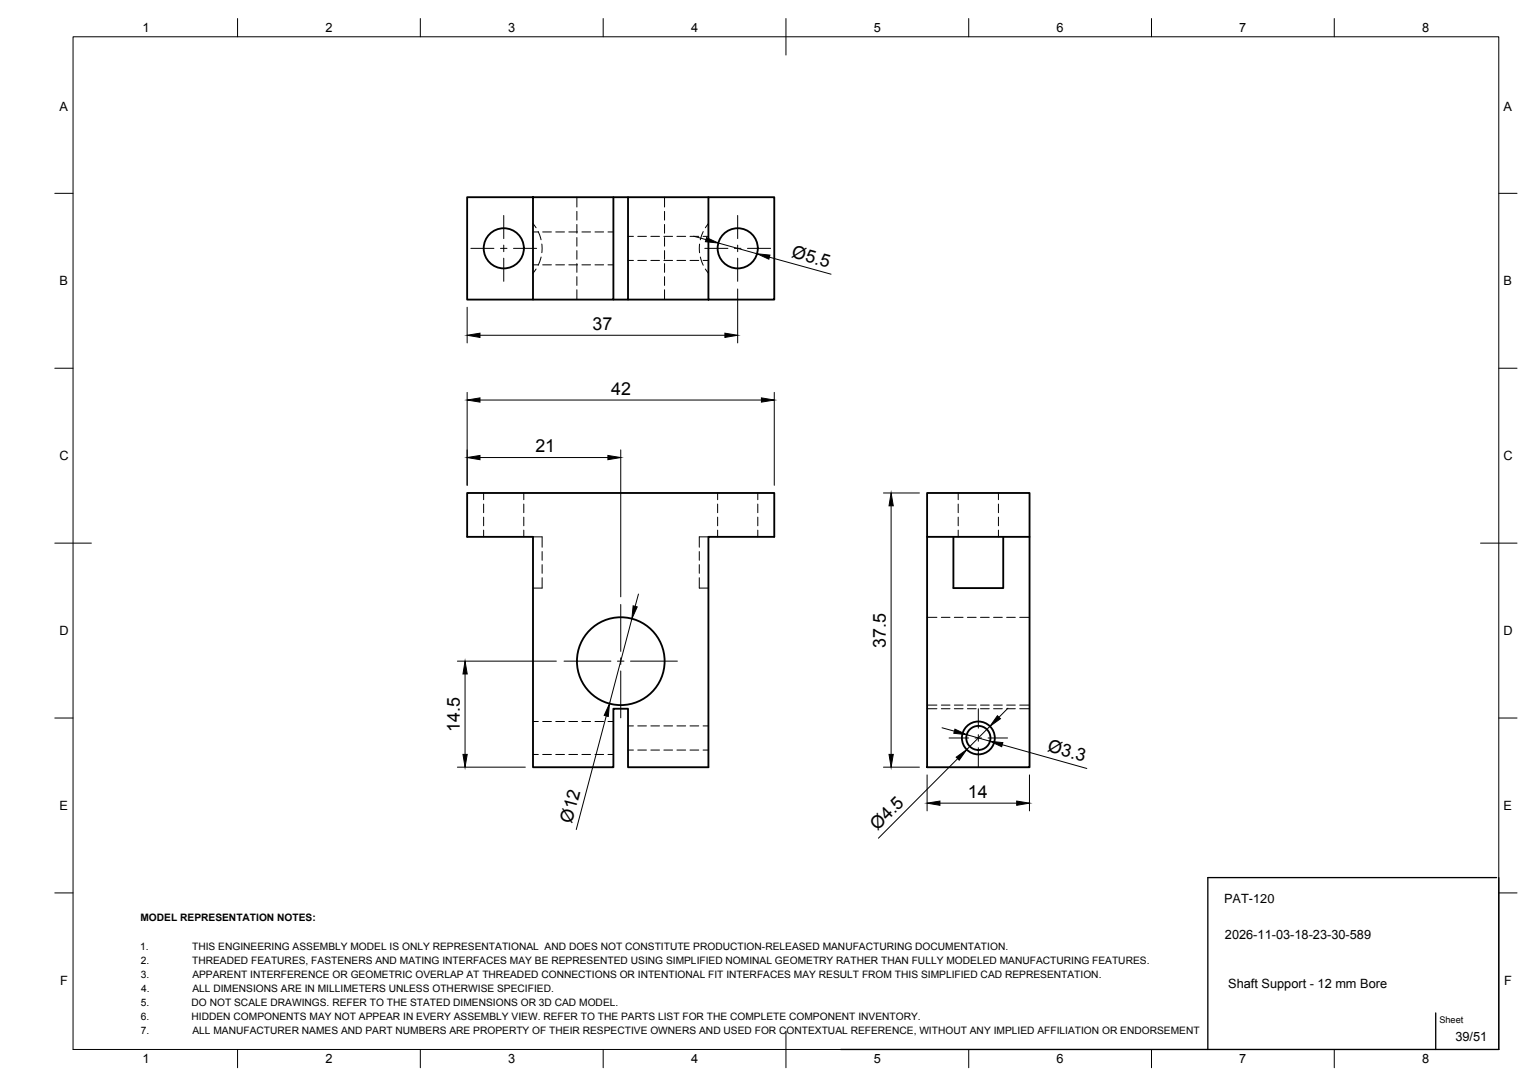
ISO-10303-21;
HEADER;
/* Generated by software containing ST-Developer
 * from STEP Tools, Inc. (www.steptools.com) 
 */

FILE_DESCRIPTION(
/* description */ ('Vibration shaker table dummy'),
/* implementation_level */ '2;1');

FILE_NAME(
/* name */ 'Shaft Support - 12 mm Bore.step',
/* time_stamp */ '2026-10-27T10:55:14-07:00',
/* author */ (''),
/* organization */ (''),
/* preprocessor_version */ 'ST-DEVELOPER v20.2',
/* originating_system */ 'Autodesk Translation Framework v15.17.0.0',
/* authorisation */ '');

FILE_SCHEMA (('AUTOMOTIVE_DESIGN { 1 0 10303 214 3 1 1 }'));
ENDSEC;

DATA;
#10=MECHANICAL_DESIGN_GEOMETRIC_PRESENTATION_REPRESENTATION('',(#720),#22394);
#628=SHAPE_REPRESENTATION_RELATIONSHIP('SRR','None',#22674,#674);
#674=ADVANCED_BREP_SHAPE_REPRESENTATION('',(#766),#22380);
#720=STYLED_ITEM('',(#22961),#766);
#766=MANIFOLD_SOLID_BREP('Body1',#9238);
#947=FACE_BOUND('',#2313,.T.);
#948=FACE_BOUND('',#2315,.T.);
#949=FACE_BOUND('',#2317,.T.);
#950=FACE_BOUND('',#2324,.T.);
#951=FACE_BOUND('',#2327,.T.);
#952=FACE_BOUND('',#2328,.T.);
#953=FACE_BOUND('',#2331,.T.);
#954=FACE_BOUND('',#2334,.T.);
#955=FACE_BOUND('',#2337,.T.);
#956=FACE_BOUND('',#2340,.T.);
#1234=PLANE('',#10350);
#1235=PLANE('',#10357);
#1236=PLANE('',#10358);
#1237=PLANE('',#10360);
#1238=PLANE('',#10362);
#1239=PLANE('',#10376);
#1240=PLANE('',#10377);
#1241=PLANE('',#10378);
#1242=PLANE('',#10379);
#1243=PLANE('',#10380);
#1244=PLANE('',#10381);
#1245=PLANE('',#10382);
#1246=PLANE('',#10383);
#1247=PLANE('',#10384);
#1248=PLANE('',#10385);
#1249=PLANE('',#10386);
#1638=FACE_OUTER_BOUND('',#2308,.T.);
#1639=FACE_OUTER_BOUND('',#2309,.T.);
#1640=FACE_OUTER_BOUND('',#2310,.T.);
#1641=FACE_OUTER_BOUND('',#2311,.T.);
#1642=FACE_OUTER_BOUND('',#2312,.T.);
#1643=FACE_OUTER_BOUND('',#2314,.T.);
#1644=FACE_OUTER_BOUND('',#2316,.T.);
#1645=FACE_OUTER_BOUND('',#2318,.T.);
#1646=FACE_OUTER_BOUND('',#2319,.T.);
#1647=FACE_OUTER_BOUND('',#2320,.T.);
#1648=FACE_OUTER_BOUND('',#2321,.T.);
#1649=FACE_OUTER_BOUND('',#2322,.T.);
#1650=FACE_OUTER_BOUND('',#2323,.T.);
#1651=FACE_OUTER_BOUND('',#2325,.T.);
#1652=FACE_OUTER_BOUND('',#2326,.T.);
#1653=FACE_OUTER_BOUND('',#2329,.T.);
#1654=FACE_OUTER_BOUND('',#2330,.T.);
#1655=FACE_OUTER_BOUND('',#2332,.T.);
#1656=FACE_OUTER_BOUND('',#2333,.T.);
#1657=FACE_OUTER_BOUND('',#2335,.T.);
#1658=FACE_OUTER_BOUND('',#2336,.T.);
#1659=FACE_OUTER_BOUND('',#2338,.T.);
#1660=FACE_OUTER_BOUND('',#2339,.T.);
#2308=EDGE_LOOP('',(#7508,#7509));
#2309=EDGE_LOOP('',(#7510,#7511,#7512,#7513));
#2310=EDGE_LOOP('',(#7514,#7515,#7516,#7517));
#2311=EDGE_LOOP('',(#7518,#7519));
#2312=EDGE_LOOP('',(#7520,#7521,#7522,#7523,#7524,#7525));
#2313=EDGE_LOOP('',(#7526));
#2314=EDGE_LOOP('',(#7527,#7528,#7529,#7530,#7531,#7532,#7533,#7534));
#2315=EDGE_LOOP('',(#7535));
#2316=EDGE_LOOP('',(#7536,#7537,#7538,#7539,#7540,#7541));
#2317=EDGE_LOOP('',(#7542));
#2318=EDGE_LOOP('',(#7543,#7544,#7545,#7546));
#2319=EDGE_LOOP('',(#7547,#7548,#7549,#7550));
#2320=EDGE_LOOP('',(#7551,#7552,#7553,#7554));
#2321=EDGE_LOOP('',(#7555,#7556,#7557,#7558));
#2322=EDGE_LOOP('',(#7559,#7560,#7561,#7562));
#2323=EDGE_LOOP('',(#7563,#7564,#7565,#7566,#7567,#7568,#7569,#7570,#7571,
#7572,#7573,#7574));
#2324=EDGE_LOOP('',(#7575));
#2325=EDGE_LOOP('',(#7576,#7577,#7578,#7579));
#2326=EDGE_LOOP('',(#7580,#7581,#7582,#7583));
#2327=EDGE_LOOP('',(#7584));
#2328=EDGE_LOOP('',(#7585));
#2329=EDGE_LOOP('',(#7586,#7587,#7588,#7589));
#2330=EDGE_LOOP('',(#7590,#7591,#7592,#7593,#7594,#7595,#7596,#7597));
#2331=EDGE_LOOP('',(#7598));
#2332=EDGE_LOOP('',(#7599,#7600,#7601,#7602));
#2333=EDGE_LOOP('',(#7603,#7604,#7605,#7606));
#2334=EDGE_LOOP('',(#7607));
#2335=EDGE_LOOP('',(#7608,#7609,#7610,#7611));
#2336=EDGE_LOOP('',(#7612,#7613,#7614,#7615));
#2337=EDGE_LOOP('',(#7616));
#2338=EDGE_LOOP('',(#7617,#7618,#7619,#7620));
#2339=EDGE_LOOP('',(#7621,#7622,#7623,#7624,#7625,#7626,#7627,#7628,#7629,
#7630,#7631,#7632));
#2340=EDGE_LOOP('',(#7633));
#2989=LINE('',#21115,#3608);
#2990=LINE('',#21119,#3609);
#2991=LINE('',#21122,#3610);
#2992=LINE('',#21126,#3611);
#2993=LINE('',#21130,#3612);
#2994=LINE('',#21133,#3613);
#2995=LINE('',#21136,#3614);
#2996=LINE('',#21138,#3615);
#2997=LINE('',#21140,#3616);
#2998=LINE('',#21142,#3617);
#2999=LINE('',#21143,#3618);
#3000=LINE('',#21148,#3619);
#3001=LINE('',#21150,#3620);
#3002=LINE('',#21151,#3621);
#3003=LINE('',#21157,#3622);
#3004=LINE('',#21159,#3623);
#3005=LINE('',#21160,#3624);
#3006=LINE('',#21162,#3625);
#3007=LINE('',#21163,#3626);
#3008=LINE('',#21170,#3627);
#3009=LINE('',#21174,#3628);
#3010=LINE('',#21179,#3629);
#3011=LINE('',#21183,#3630);
#3012=LINE('',#21188,#3631);
#3013=LINE('',#21192,#3632);
#3014=LINE('',#21194,#3633);
#3015=LINE('',#21195,#3634);
#3016=LINE('',#21197,#3635);
#3017=LINE('',#21199,#3636);
#3018=LINE('',#21201,#3637);
#3019=LINE('',#21203,#3638);
#3020=LINE('',#21205,#3639);
#3021=LINE('',#21206,#3640);
#3022=LINE('',#21209,#3641);
#3023=LINE('',#21210,#3642);
#3024=LINE('',#21213,#3643);
#3025=LINE('',#21214,#3644);
#3026=LINE('',#21216,#3645);
#3027=LINE('',#21219,#3646);
#3028=LINE('',#21220,#3647);
#3029=LINE('',#21223,#3648);
#3030=LINE('',#21224,#3649);
#3031=LINE('',#21227,#3650);
#3032=LINE('',#21228,#3651);
#3033=LINE('',#21231,#3652);
#3034=LINE('',#21232,#3653);
#3035=LINE('',#21235,#3654);
#3036=LINE('',#21236,#3655);
#3037=LINE('',#21238,#3656);
#3608=VECTOR('',#12499,1.);
#3609=VECTOR('',#12504,1.);
#3610=VECTOR('',#12507,1.);
#3611=VECTOR('',#12510,1.);
#3612=VECTOR('',#12513,1.);
#3613=VECTOR('',#12518,1.);
#3614=VECTOR('',#12521,1.);
#3615=VECTOR('',#12522,1.);
#3616=VECTOR('',#12523,1.);
#3617=VECTOR('',#12524,1.);
#3618=VECTOR('',#12525,1.);
#3619=VECTOR('',#12530,1.);
#3620=VECTOR('',#12531,1.);
#3621=VECTOR('',#12532,1.);
#3622=VECTOR('',#12537,1.);
#3623=VECTOR('',#12538,1.);
#3624=VECTOR('',#12539,1.);
#3625=VECTOR('',#12540,1.);
#3626=VECTOR('',#12541,1.);
#3627=VECTOR('',#12548,0.225);
#3628=VECTOR('',#12553,0.165);
#3629=VECTOR('',#12560,0.275);
#3630=VECTOR('',#12565,0.275);
#3631=VECTOR('',#12570,0.6);
#3632=VECTOR('',#12575,1.);
#3633=VECTOR('',#12576,1.);
#3634=VECTOR('',#12577,1.);
#3635=VECTOR('',#12578,1.);
#3636=VECTOR('',#12579,1.);
#3637=VECTOR('',#12580,1.);
#3638=VECTOR('',#12581,1.);
#3639=VECTOR('',#12582,1.);
#3640=VECTOR('',#12583,1.);
#3641=VECTOR('',#12586,1.);
#3642=VECTOR('',#12587,1.);
#3643=VECTOR('',#12590,1.);
#3644=VECTOR('',#12591,1.);
#3645=VECTOR('',#12594,1.);
#3646=VECTOR('',#12597,1.);
#3647=VECTOR('',#12598,1.);
#3648=VECTOR('',#12601,1.);
#3649=VECTOR('',#12602,1.);
#3650=VECTOR('',#12605,1.);
#3651=VECTOR('',#12606,1.);
#3652=VECTOR('',#12609,1.);
#3653=VECTOR('',#12610,1.);
#3654=VECTOR('',#12613,1.);
#3655=VECTOR('',#12614,1.);
#3656=VECTOR('',#12617,1.);
#4120=CIRCLE('',#10351,0.525);
#4121=CIRCLE('',#10353,0.525);
#4122=CIRCLE('',#10355,0.525);
#4123=CIRCLE('',#10356,0.525);
#4124=CIRCLE('',#10359,0.275);
#4125=CIRCLE('',#10361,0.165);
#4126=CIRCLE('',#10363,0.275);
#4127=CIRCLE('',#10365,0.225);
#4128=CIRCLE('',#10366,0.225);
#4129=CIRCLE('',#10368,0.165);
#4130=CIRCLE('',#10370,0.275);
#4131=CIRCLE('',#10372,0.275);
#4132=CIRCLE('',#10374,0.6);
#4133=CIRCLE('',#10375,0.6);
#4787=VERTEX_POINT('',#21113);
#4788=VERTEX_POINT('',#21114);
#4789=VERTEX_POINT('',#21118);
#4790=VERTEX_POINT('',#21120);
#4791=VERTEX_POINT('',#21124);
#4792=VERTEX_POINT('',#21125);
#4793=VERTEX_POINT('',#21127);
#4794=VERTEX_POINT('',#21129);
#4795=VERTEX_POINT('',#21135);
#4796=VERTEX_POINT('',#21137);
#4797=VERTEX_POINT('',#21139);
#4798=VERTEX_POINT('',#21141);
#4799=VERTEX_POINT('',#21144);
#4800=VERTEX_POINT('',#21147);
#4801=VERTEX_POINT('',#21149);
#4802=VERTEX_POINT('',#21152);
#4803=VERTEX_POINT('',#21155);
#4804=VERTEX_POINT('',#21156);
#4805=VERTEX_POINT('',#21158);
#4806=VERTEX_POINT('',#21161);
#4807=VERTEX_POINT('',#21164);
#4808=VERTEX_POINT('',#21167);
#4809=VERTEX_POINT('',#21169);
#4810=VERTEX_POINT('',#21173);
#4811=VERTEX_POINT('',#21177);
#4812=VERTEX_POINT('',#21181);
#4813=VERTEX_POINT('',#21185);
#4814=VERTEX_POINT('',#21187);
#4815=VERTEX_POINT('',#21191);
#4816=VERTEX_POINT('',#21193);
#4817=VERTEX_POINT('',#21196);
#4818=VERTEX_POINT('',#21198);
#4819=VERTEX_POINT('',#21200);
#4820=VERTEX_POINT('',#21202);
#4821=VERTEX_POINT('',#21204);
#4822=VERTEX_POINT('',#21208);
#4823=VERTEX_POINT('',#21212);
#4824=VERTEX_POINT('',#21218);
#4825=VERTEX_POINT('',#21222);
#4826=VERTEX_POINT('',#21226);
#4827=VERTEX_POINT('',#21230);
#4828=VERTEX_POINT('',#21234);
#5747=EDGE_CURVE('',#4787,#4788,#2989,.T.);
#5748=EDGE_CURVE('',#4788,#4787,#4120,.T.);
#5749=EDGE_CURVE('',#4789,#4787,#2990,.T.);
#5750=EDGE_CURVE('',#4790,#4789,#4121,.T.);
#5751=EDGE_CURVE('',#4788,#4790,#2991,.T.);
#5752=EDGE_CURVE('',#4791,#4792,#2992,.T.);
#5753=EDGE_CURVE('',#4791,#4793,#4122,.T.);
#5754=EDGE_CURVE('',#4794,#4793,#2993,.T.);
#5755=EDGE_CURVE('',#4792,#4794,#4123,.T.);
#5756=EDGE_CURVE('',#4793,#4791,#2994,.T.);
#5757=EDGE_CURVE('',#4789,#4795,#2995,.T.);
#5758=EDGE_CURVE('',#4796,#4795,#2996,.T.);
#5759=EDGE_CURVE('',#4796,#4797,#2997,.T.);
#5760=EDGE_CURVE('',#4798,#4797,#2998,.T.);
#5761=EDGE_CURVE('',#4798,#4790,#2999,.T.);
#5762=EDGE_CURVE('',#4799,#4799,#4124,.T.);
#5763=EDGE_CURVE('',#4800,#4798,#3000,.T.);
#5764=EDGE_CURVE('',#4800,#4801,#3001,.T.);
#5765=EDGE_CURVE('',#4795,#4801,#3002,.T.);
#5766=EDGE_CURVE('',#4802,#4802,#4125,.T.);
#5767=EDGE_CURVE('',#4803,#4804,#3003,.T.);
#5768=EDGE_CURVE('',#4805,#4804,#3004,.T.);
#5769=EDGE_CURVE('',#4792,#4805,#3005,.T.);
#5770=EDGE_CURVE('',#4806,#4794,#3006,.T.);
#5771=EDGE_CURVE('',#4803,#4806,#3007,.T.);
#5772=EDGE_CURVE('',#4807,#4807,#4126,.T.);
#5773=EDGE_CURVE('',#4808,#4808,#4127,.T.);
#5774=EDGE_CURVE('',#4808,#4809,#3008,.T.);
#5775=EDGE_CURVE('',#4809,#4809,#4128,.T.);
#5776=EDGE_CURVE('',#4802,#4810,#3009,.T.);
#5777=EDGE_CURVE('',#4810,#4810,#4129,.T.);
#5778=EDGE_CURVE('',#4811,#4811,#4130,.T.);
#5779=EDGE_CURVE('',#4811,#4799,#3010,.T.);
#5780=EDGE_CURVE('',#4812,#4812,#4131,.T.);
#5781=EDGE_CURVE('',#4812,#4807,#3011,.T.);
#5782=EDGE_CURVE('',#4813,#4813,#4132,.T.);
#5783=EDGE_CURVE('',#4813,#4814,#3012,.T.);
#5784=EDGE_CURVE('',#4814,#4814,#4133,.T.);
#5785=EDGE_CURVE('',#4797,#4815,#3013,.T.);
#5786=EDGE_CURVE('',#4815,#4816,#3014,.T.);
#5787=EDGE_CURVE('',#4816,#4803,#3015,.T.);
#5788=EDGE_CURVE('',#4806,#4817,#3016,.T.);
#5789=EDGE_CURVE('',#4817,#4818,#3017,.T.);
#5790=EDGE_CURVE('',#4818,#4819,#3018,.T.);
#5791=EDGE_CURVE('',#4819,#4820,#3019,.T.);
#5792=EDGE_CURVE('',#4820,#4821,#3020,.T.);
#5793=EDGE_CURVE('',#4821,#4800,#3021,.T.);
#5794=EDGE_CURVE('',#4822,#4796,#3022,.T.);
#5795=EDGE_CURVE('',#4815,#4822,#3023,.T.);
#5796=EDGE_CURVE('',#4823,#4822,#3024,.T.);
#5797=EDGE_CURVE('',#4816,#4823,#3025,.T.);
#5798=EDGE_CURVE('',#4804,#4823,#3026,.T.);
#5799=EDGE_CURVE('',#4824,#4805,#3027,.T.);
#5800=EDGE_CURVE('',#4817,#4824,#3028,.T.);
#5801=EDGE_CURVE('',#4825,#4824,#3029,.T.);
#5802=EDGE_CURVE('',#4818,#4825,#3030,.T.);
#5803=EDGE_CURVE('',#4826,#4825,#3031,.T.);
#5804=EDGE_CURVE('',#4819,#4826,#3032,.T.);
#5805=EDGE_CURVE('',#4827,#4826,#3033,.T.);
#5806=EDGE_CURVE('',#4820,#4827,#3034,.T.);
#5807=EDGE_CURVE('',#4828,#4827,#3035,.T.);
#5808=EDGE_CURVE('',#4821,#4828,#3036,.T.);
#5809=EDGE_CURVE('',#4801,#4828,#3037,.T.);
#7508=ORIENTED_EDGE('',*,*,#5747,.F.);
#7509=ORIENTED_EDGE('',*,*,#5748,.F.);
#7510=ORIENTED_EDGE('',*,*,#5749,.F.);
#7511=ORIENTED_EDGE('',*,*,#5750,.F.);
#7512=ORIENTED_EDGE('',*,*,#5751,.F.);
#7513=ORIENTED_EDGE('',*,*,#5748,.T.);
#7514=ORIENTED_EDGE('',*,*,#5752,.F.);
#7515=ORIENTED_EDGE('',*,*,#5753,.T.);
#7516=ORIENTED_EDGE('',*,*,#5754,.F.);
#7517=ORIENTED_EDGE('',*,*,#5755,.F.);
#7518=ORIENTED_EDGE('',*,*,#5756,.F.);
#7519=ORIENTED_EDGE('',*,*,#5753,.F.);
#7520=ORIENTED_EDGE('',*,*,#5757,.T.);
#7521=ORIENTED_EDGE('',*,*,#5758,.F.);
#7522=ORIENTED_EDGE('',*,*,#5759,.T.);
#7523=ORIENTED_EDGE('',*,*,#5760,.F.);
#7524=ORIENTED_EDGE('',*,*,#5761,.T.);
#7525=ORIENTED_EDGE('',*,*,#5750,.T.);
#7526=ORIENTED_EDGE('',*,*,#5762,.T.);
#7527=ORIENTED_EDGE('',*,*,#5749,.T.);
#7528=ORIENTED_EDGE('',*,*,#5747,.T.);
#7529=ORIENTED_EDGE('',*,*,#5751,.T.);
#7530=ORIENTED_EDGE('',*,*,#5761,.F.);
#7531=ORIENTED_EDGE('',*,*,#5763,.F.);
#7532=ORIENTED_EDGE('',*,*,#5764,.T.);
#7533=ORIENTED_EDGE('',*,*,#5765,.F.);
#7534=ORIENTED_EDGE('',*,*,#5757,.F.);
#7535=ORIENTED_EDGE('',*,*,#5766,.T.);
#7536=ORIENTED_EDGE('',*,*,#5767,.T.);
#7537=ORIENTED_EDGE('',*,*,#5768,.F.);
#7538=ORIENTED_EDGE('',*,*,#5769,.F.);
#7539=ORIENTED_EDGE('',*,*,#5755,.T.);
#7540=ORIENTED_EDGE('',*,*,#5770,.F.);
#7541=ORIENTED_EDGE('',*,*,#5771,.F.);
#7542=ORIENTED_EDGE('',*,*,#5772,.T.);
#7543=ORIENTED_EDGE('',*,*,#5773,.F.);
#7544=ORIENTED_EDGE('',*,*,#5774,.T.);
#7545=ORIENTED_EDGE('',*,*,#5775,.F.);
#7546=ORIENTED_EDGE('',*,*,#5774,.F.);
#7547=ORIENTED_EDGE('',*,*,#5766,.F.);
#7548=ORIENTED_EDGE('',*,*,#5776,.T.);
#7549=ORIENTED_EDGE('',*,*,#5777,.F.);
#7550=ORIENTED_EDGE('',*,*,#5776,.F.);
#7551=ORIENTED_EDGE('',*,*,#5778,.F.);
#7552=ORIENTED_EDGE('',*,*,#5779,.T.);
#7553=ORIENTED_EDGE('',*,*,#5762,.F.);
#7554=ORIENTED_EDGE('',*,*,#5779,.F.);
#7555=ORIENTED_EDGE('',*,*,#5780,.F.);
#7556=ORIENTED_EDGE('',*,*,#5781,.T.);
#7557=ORIENTED_EDGE('',*,*,#5772,.F.);
#7558=ORIENTED_EDGE('',*,*,#5781,.F.);
#7559=ORIENTED_EDGE('',*,*,#5782,.F.);
#7560=ORIENTED_EDGE('',*,*,#5783,.T.);
#7561=ORIENTED_EDGE('',*,*,#5784,.F.);
#7562=ORIENTED_EDGE('',*,*,#5783,.F.);
#7563=ORIENTED_EDGE('',*,*,#5760,.T.);
#7564=ORIENTED_EDGE('',*,*,#5785,.T.);
#7565=ORIENTED_EDGE('',*,*,#5786,.T.);
#7566=ORIENTED_EDGE('',*,*,#5787,.T.);
#7567=ORIENTED_EDGE('',*,*,#5771,.T.);
#7568=ORIENTED_EDGE('',*,*,#5788,.T.);
#7569=ORIENTED_EDGE('',*,*,#5789,.T.);
#7570=ORIENTED_EDGE('',*,*,#5790,.T.);
#7571=ORIENTED_EDGE('',*,*,#5791,.T.);
#7572=ORIENTED_EDGE('',*,*,#5792,.T.);
#7573=ORIENTED_EDGE('',*,*,#5793,.T.);
#7574=ORIENTED_EDGE('',*,*,#5763,.T.);
#7575=ORIENTED_EDGE('',*,*,#5782,.T.);
#7576=ORIENTED_EDGE('',*,*,#5759,.F.);
#7577=ORIENTED_EDGE('',*,*,#5794,.F.);
#7578=ORIENTED_EDGE('',*,*,#5795,.F.);
#7579=ORIENTED_EDGE('',*,*,#5785,.F.);
#7580=ORIENTED_EDGE('',*,*,#5795,.T.);
#7581=ORIENTED_EDGE('',*,*,#5796,.F.);
#7582=ORIENTED_EDGE('',*,*,#5797,.F.);
#7583=ORIENTED_EDGE('',*,*,#5786,.F.);
#7584=ORIENTED_EDGE('',*,*,#5778,.T.);
#7585=ORIENTED_EDGE('',*,*,#5780,.T.);
#7586=ORIENTED_EDGE('',*,*,#5797,.T.);
#7587=ORIENTED_EDGE('',*,*,#5798,.F.);
#7588=ORIENTED_EDGE('',*,*,#5767,.F.);
#7589=ORIENTED_EDGE('',*,*,#5787,.F.);
#7590=ORIENTED_EDGE('',*,*,#5752,.T.);
#7591=ORIENTED_EDGE('',*,*,#5769,.T.);
#7592=ORIENTED_EDGE('',*,*,#5799,.F.);
#7593=ORIENTED_EDGE('',*,*,#5800,.F.);
#7594=ORIENTED_EDGE('',*,*,#5788,.F.);
#7595=ORIENTED_EDGE('',*,*,#5770,.T.);
#7596=ORIENTED_EDGE('',*,*,#5754,.T.);
#7597=ORIENTED_EDGE('',*,*,#5756,.T.);
#7598=ORIENTED_EDGE('',*,*,#5775,.T.);
#7599=ORIENTED_EDGE('',*,*,#5800,.T.);
#7600=ORIENTED_EDGE('',*,*,#5801,.F.);
#7601=ORIENTED_EDGE('',*,*,#5802,.F.);
#7602=ORIENTED_EDGE('',*,*,#5789,.F.);
#7603=ORIENTED_EDGE('',*,*,#5802,.T.);
#7604=ORIENTED_EDGE('',*,*,#5803,.F.);
#7605=ORIENTED_EDGE('',*,*,#5804,.F.);
#7606=ORIENTED_EDGE('',*,*,#5790,.F.);
#7607=ORIENTED_EDGE('',*,*,#5773,.T.);
#7608=ORIENTED_EDGE('',*,*,#5804,.T.);
#7609=ORIENTED_EDGE('',*,*,#5805,.F.);
#7610=ORIENTED_EDGE('',*,*,#5806,.F.);
#7611=ORIENTED_EDGE('',*,*,#5791,.F.);
#7612=ORIENTED_EDGE('',*,*,#5806,.T.);
#7613=ORIENTED_EDGE('',*,*,#5807,.F.);
#7614=ORIENTED_EDGE('',*,*,#5808,.F.);
#7615=ORIENTED_EDGE('',*,*,#5792,.F.);
#7616=ORIENTED_EDGE('',*,*,#5777,.T.);
#7617=ORIENTED_EDGE('',*,*,#5808,.T.);
#7618=ORIENTED_EDGE('',*,*,#5809,.F.);
#7619=ORIENTED_EDGE('',*,*,#5764,.F.);
#7620=ORIENTED_EDGE('',*,*,#5793,.F.);
#7621=ORIENTED_EDGE('',*,*,#5758,.T.);
#7622=ORIENTED_EDGE('',*,*,#5765,.T.);
#7623=ORIENTED_EDGE('',*,*,#5809,.T.);
#7624=ORIENTED_EDGE('',*,*,#5807,.T.);
#7625=ORIENTED_EDGE('',*,*,#5805,.T.);
#7626=ORIENTED_EDGE('',*,*,#5803,.T.);
#7627=ORIENTED_EDGE('',*,*,#5801,.T.);
#7628=ORIENTED_EDGE('',*,*,#5799,.T.);
#7629=ORIENTED_EDGE('',*,*,#5768,.T.);
#7630=ORIENTED_EDGE('',*,*,#5798,.T.);
#7631=ORIENTED_EDGE('',*,*,#5796,.T.);
#7632=ORIENTED_EDGE('',*,*,#5794,.T.);
#7633=ORIENTED_EDGE('',*,*,#5784,.T.);
#8623=CYLINDRICAL_SURFACE('',#10352,0.525);
#8624=CYLINDRICAL_SURFACE('',#10354,0.525);
#8625=CYLINDRICAL_SURFACE('',#10364,0.225);
#8626=CYLINDRICAL_SURFACE('',#10367,0.165);
#8627=CYLINDRICAL_SURFACE('',#10369,0.275);
#8628=CYLINDRICAL_SURFACE('',#10371,0.275);
#8629=CYLINDRICAL_SURFACE('',#10373,0.6);
#9003=ADVANCED_FACE('',(#1638),#1234,.F.);
#9004=ADVANCED_FACE('',(#1639),#8623,.F.);
#9005=ADVANCED_FACE('',(#1640),#8624,.F.);
#9006=ADVANCED_FACE('',(#1641),#1235,.F.);
#9007=ADVANCED_FACE('',(#1642,#947),#1236,.T.);
#9008=ADVANCED_FACE('',(#1643,#948),#1237,.T.);
#9009=ADVANCED_FACE('',(#1644,#949),#1238,.T.);
#9010=ADVANCED_FACE('',(#1645),#8625,.F.);
#9011=ADVANCED_FACE('',(#1646),#8626,.F.);
#9012=ADVANCED_FACE('',(#1647),#8627,.F.);
#9013=ADVANCED_FACE('',(#1648),#8628,.F.);
#9014=ADVANCED_FACE('',(#1649),#8629,.F.);
#9015=ADVANCED_FACE('',(#1650,#950),#1239,.T.);
#9016=ADVANCED_FACE('',(#1651),#1240,.T.);
#9017=ADVANCED_FACE('',(#1652,#951,#952),#1241,.T.);
#9018=ADVANCED_FACE('',(#1653),#1242,.T.);
#9019=ADVANCED_FACE('',(#1654,#953),#1243,.T.);
#9020=ADVANCED_FACE('',(#1655),#1244,.T.);
#9021=ADVANCED_FACE('',(#1656,#954),#1245,.T.);
#9022=ADVANCED_FACE('',(#1657),#1246,.T.);
#9023=ADVANCED_FACE('',(#1658,#955),#1247,.T.);
#9024=ADVANCED_FACE('',(#1659),#1248,.T.);
#9025=ADVANCED_FACE('',(#1660,#956),#1249,.T.);
#9238=CLOSED_SHELL('',(#9003,#9004,#9005,#9006,#9007,#9008,#9009,#9010,
#9011,#9012,#9013,#9014,#9015,#9016,#9017,#9018,#9019,#9020,#9021,#9022,
#9023,#9024,#9025));
#10349=AXIS2_PLACEMENT_3D('',#21111,#12495,#12496);
#10350=AXIS2_PLACEMENT_3D('',#21112,#12497,#12498);
#10351=AXIS2_PLACEMENT_3D('',#21116,#12500,#12501);
#10352=AXIS2_PLACEMENT_3D('',#21117,#12502,#12503);
#10353=AXIS2_PLACEMENT_3D('',#21121,#12505,#12506);
#10354=AXIS2_PLACEMENT_3D('',#21123,#12508,#12509);
#10355=AXIS2_PLACEMENT_3D('',#21128,#12511,#12512);
#10356=AXIS2_PLACEMENT_3D('',#21131,#12514,#12515);
#10357=AXIS2_PLACEMENT_3D('',#21132,#12516,#12517);
#10358=AXIS2_PLACEMENT_3D('',#21134,#12519,#12520);
#10359=AXIS2_PLACEMENT_3D('',#21145,#12526,#12527);
#10360=AXIS2_PLACEMENT_3D('',#21146,#12528,#12529);
#10361=AXIS2_PLACEMENT_3D('',#21153,#12533,#12534);
#10362=AXIS2_PLACEMENT_3D('',#21154,#12535,#12536);
#10363=AXIS2_PLACEMENT_3D('',#21165,#12542,#12543);
#10364=AXIS2_PLACEMENT_3D('',#21166,#12544,#12545);
#10365=AXIS2_PLACEMENT_3D('',#21168,#12546,#12547);
#10366=AXIS2_PLACEMENT_3D('',#21171,#12549,#12550);
#10367=AXIS2_PLACEMENT_3D('',#21172,#12551,#12552);
#10368=AXIS2_PLACEMENT_3D('',#21175,#12554,#12555);
#10369=AXIS2_PLACEMENT_3D('',#21176,#12556,#12557);
#10370=AXIS2_PLACEMENT_3D('',#21178,#12558,#12559);
#10371=AXIS2_PLACEMENT_3D('',#21180,#12561,#12562);
#10372=AXIS2_PLACEMENT_3D('',#21182,#12563,#12564);
#10373=AXIS2_PLACEMENT_3D('',#21184,#12566,#12567);
#10374=AXIS2_PLACEMENT_3D('',#21186,#12568,#12569);
#10375=AXIS2_PLACEMENT_3D('',#21189,#12571,#12572);
#10376=AXIS2_PLACEMENT_3D('',#21190,#12573,#12574);
#10377=AXIS2_PLACEMENT_3D('',#21207,#12584,#12585);
#10378=AXIS2_PLACEMENT_3D('',#21211,#12588,#12589);
#10379=AXIS2_PLACEMENT_3D('',#21215,#12592,#12593);
#10380=AXIS2_PLACEMENT_3D('',#21217,#12595,#12596);
#10381=AXIS2_PLACEMENT_3D('',#21221,#12599,#12600);
#10382=AXIS2_PLACEMENT_3D('',#21225,#12603,#12604);
#10383=AXIS2_PLACEMENT_3D('',#21229,#12607,#12608);
#10384=AXIS2_PLACEMENT_3D('',#21233,#12611,#12612);
#10385=AXIS2_PLACEMENT_3D('',#21237,#12615,#12616);
#10386=AXIS2_PLACEMENT_3D('',#21239,#12618,#12619);
#12495=DIRECTION('axis',(0.,0.,1.));
#12496=DIRECTION('refdir',(1.,0.,0.));
#12497=DIRECTION('center_axis',(0.,0.,1.));
#12498=DIRECTION('ref_axis',(1.,0.,0.));
#12499=DIRECTION('',(0.,-1.,0.));
#12500=DIRECTION('center_axis',(0.,0.,1.));
#12501=DIRECTION('ref_axis',(1.,0.,0.));
#12502=DIRECTION('center_axis',(0.,0.,1.));
#12503=DIRECTION('ref_axis',(1.,0.,0.));
#12504=DIRECTION('',(0.,0.,1.));
#12505=DIRECTION('center_axis',(0.,0.,1.));
#12506=DIRECTION('ref_axis',(1.,0.,0.));
#12507=DIRECTION('',(0.,0.,-1.));
#12508=DIRECTION('center_axis',(0.,0.,1.));
#12509=DIRECTION('ref_axis',(-1.,1.22464679914735E-16,0.));
#12510=DIRECTION('',(0.,0.,-1.));
#12511=DIRECTION('center_axis',(0.,0.,1.));
#12512=DIRECTION('ref_axis',(1.,0.,0.));
#12513=DIRECTION('',(0.,0.,1.));
#12514=DIRECTION('center_axis',(0.,0.,1.));
#12515=DIRECTION('ref_axis',(1.,0.,0.));
#12516=DIRECTION('center_axis',(0.,0.,1.));
#12517=DIRECTION('ref_axis',(1.,0.,0.));
#12518=DIRECTION('',(0.,1.,0.));
#12519=DIRECTION('center_axis',(0.,0.,1.));
#12520=DIRECTION('ref_axis',(1.,0.,0.));
#12521=DIRECTION('',(0.,1.,0.));
#12522=DIRECTION('',(1.,0.,0.));
#12523=DIRECTION('',(0.,-1.,0.));
#12524=DIRECTION('',(-1.,0.,0.));
#12525=DIRECTION('',(0.,1.,0.));
#12526=DIRECTION('center_axis',(0.,0.,-1.));
#12527=DIRECTION('ref_axis',(1.,0.,0.));
#12528=DIRECTION('center_axis',(-1.,0.,0.));
#12529=DIRECTION('ref_axis',(0.,0.,1.));
#12530=DIRECTION('',(0.,0.,-1.));
#12531=DIRECTION('',(0.,1.,0.));
#12532=DIRECTION('',(0.,0.,1.));
#12533=DIRECTION('center_axis',(1.,0.,0.));
#12534=DIRECTION('ref_axis',(0.,0.,-1.));
#12535=DIRECTION('center_axis',(0.,0.,1.));
#12536=DIRECTION('ref_axis',(1.,0.,0.));
#12537=DIRECTION('',(0.,1.,0.));
#12538=DIRECTION('',(1.,0.,0.));
#12539=DIRECTION('',(0.,1.,0.));
#12540=DIRECTION('',(0.,1.,0.));
#12541=DIRECTION('',(-1.,0.,0.));
#12542=DIRECTION('center_axis',(0.,0.,-1.));
#12543=DIRECTION('ref_axis',(1.,0.,0.));
#12544=DIRECTION('center_axis',(1.,0.,0.));
#12545=DIRECTION('ref_axis',(0.,0.,-1.));
#12546=DIRECTION('center_axis',(1.,0.,0.));
#12547=DIRECTION('ref_axis',(0.,0.,-1.));
#12548=DIRECTION('',(1.,0.,0.));
#12549=DIRECTION('center_axis',(-1.,0.,0.));
#12550=DIRECTION('ref_axis',(0.,0.,-1.));
#12551=DIRECTION('center_axis',(1.,0.,0.));
#12552=DIRECTION('ref_axis',(0.,0.,-1.));
#12553=DIRECTION('',(1.,0.,0.));
#12554=DIRECTION('center_axis',(-1.,0.,0.));
#12555=DIRECTION('ref_axis',(0.,0.,-1.));
#12556=DIRECTION('center_axis',(0.,0.,1.));
#12557=DIRECTION('ref_axis',(1.,0.,0.));
#12558=DIRECTION('center_axis',(0.,0.,1.));
#12559=DIRECTION('ref_axis',(1.,0.,0.));
#12560=DIRECTION('',(0.,0.,1.));
#12561=DIRECTION('center_axis',(0.,0.,1.));
#12562=DIRECTION('ref_axis',(1.,0.,0.));
#12563=DIRECTION('center_axis',(0.,0.,1.));
#12564=DIRECTION('ref_axis',(1.,0.,0.));
#12565=DIRECTION('',(0.,0.,1.));
#12566=DIRECTION('center_axis',(0.,1.,0.));
#12567=DIRECTION('ref_axis',(1.,0.,0.));
#12568=DIRECTION('center_axis',(0.,1.,0.));
#12569=DIRECTION('ref_axis',(1.,0.,0.));
#12570=DIRECTION('',(0.,1.,0.));
#12571=DIRECTION('center_axis',(0.,-1.,0.));
#12572=DIRECTION('ref_axis',(1.,0.,0.));
#12573=DIRECTION('center_axis',(0.,-1.,0.));
#12574=DIRECTION('ref_axis',(0.,0.,-1.));
#12575=DIRECTION('',(0.,0.,-1.));
#12576=DIRECTION('',(1.,0.,0.));
#12577=DIRECTION('',(0.,0.,1.));
#12578=DIRECTION('',(0.,0.,1.));
#12579=DIRECTION('',(-1.,0.,0.));
#12580=DIRECTION('',(0.,0.,-1.));
#12581=DIRECTION('',(-1.,0.,0.));
#12582=DIRECTION('',(0.,0.,1.));
#12583=DIRECTION('',(-1.,0.,0.));
#12584=DIRECTION('center_axis',(-1.,0.,0.));
#12585=DIRECTION('ref_axis',(0.,0.,1.));
#12586=DIRECTION('',(0.,0.,1.));
#12587=DIRECTION('',(0.,1.,0.));
#12588=DIRECTION('center_axis',(0.,0.,-1.));
#12589=DIRECTION('ref_axis',(-1.,0.,0.));
#12590=DIRECTION('',(-1.,0.,0.));
#12591=DIRECTION('',(0.,1.,0.));
#12592=DIRECTION('center_axis',(1.,0.,0.));
#12593=DIRECTION('ref_axis',(0.,0.,-1.));
#12594=DIRECTION('',(0.,0.,-1.));
#12595=DIRECTION('center_axis',(1.,0.,0.));
#12596=DIRECTION('ref_axis',(0.,0.,-1.));
#12597=DIRECTION('',(0.,0.,-1.));
#12598=DIRECTION('',(0.,1.,0.));
#12599=DIRECTION('center_axis',(0.,0.,1.));
#12600=DIRECTION('ref_axis',(1.,0.,0.));
#12601=DIRECTION('',(1.,0.,0.));
#12602=DIRECTION('',(0.,1.,0.));
#12603=DIRECTION('center_axis',(-1.,0.,0.));
#12604=DIRECTION('ref_axis',(0.,0.,1.));
#12605=DIRECTION('',(0.,0.,1.));
#12606=DIRECTION('',(0.,1.,0.));
#12607=DIRECTION('center_axis',(0.,0.,1.));
#12608=DIRECTION('ref_axis',(1.,0.,0.));
#12609=DIRECTION('',(1.,0.,0.));
#12610=DIRECTION('',(0.,1.,0.));
#12611=DIRECTION('center_axis',(1.,0.,0.));
#12612=DIRECTION('ref_axis',(0.,0.,-1.));
#12613=DIRECTION('',(0.,0.,-1.));
#12614=DIRECTION('',(0.,1.,0.));
#12615=DIRECTION('center_axis',(0.,0.,1.));
#12616=DIRECTION('ref_axis',(1.,0.,0.));
#12617=DIRECTION('',(1.,0.,0.));
#12618=DIRECTION('center_axis',(0.,1.,0.));
#12619=DIRECTION('ref_axis',(0.,0.,1.));
#21111=CARTESIAN_POINT('',(0.,0.,0.));
#21112=CARTESIAN_POINT('Origin',(-1.6,0.,1.3));
#21113=CARTESIAN_POINT('',(-1.2,0.340036762718386,1.3));
#21114=CARTESIAN_POINT('',(-1.2,-0.340036762718386,1.3));
#21115=CARTESIAN_POINT('',(-1.2,0.,1.3));
#21116=CARTESIAN_POINT('Origin',(-1.6,0.,1.3));
#21117=CARTESIAN_POINT('Origin',(-1.6,0.,0.6));
#21118=CARTESIAN_POINT('',(-1.2,0.340036762718386,0.6));
#21119=CARTESIAN_POINT('',(-1.2,0.340036762718386,0.6));
#21120=CARTESIAN_POINT('',(-1.2,-0.340036762718386,0.6));
#21121=CARTESIAN_POINT('Origin',(-1.6,0.,0.6));
#21122=CARTESIAN_POINT('',(-1.2,-0.340036762718386,0.6));
#21123=CARTESIAN_POINT('Origin',(1.6,0.,0.6));
#21124=CARTESIAN_POINT('',(1.2,0.340036762718386,1.3));
#21125=CARTESIAN_POINT('',(1.2,0.340036762718386,0.6));
#21126=CARTESIAN_POINT('',(1.2,0.340036762718386,0.6));
#21127=CARTESIAN_POINT('',(1.2,-0.340036762718386,1.3));
#21128=CARTESIAN_POINT('Origin',(1.6,0.,1.3));
#21129=CARTESIAN_POINT('',(1.2,-0.340036762718386,0.6));
#21130=CARTESIAN_POINT('',(1.2,-0.340036762718386,0.6));
#21131=CARTESIAN_POINT('Origin',(1.6,0.,0.6));
#21132=CARTESIAN_POINT('Origin',(1.6,0.,1.3));
#21133=CARTESIAN_POINT('',(1.2,0.,1.3));
#21134=CARTESIAN_POINT('Origin',(-2.1,0.,0.6));
#21135=CARTESIAN_POINT('',(-1.2,0.7,0.6));
#21136=CARTESIAN_POINT('',(-1.2,0.,0.6));
#21137=CARTESIAN_POINT('',(-2.1,0.7,0.6));
#21138=CARTESIAN_POINT('',(-1.2,0.7,0.6));
#21139=CARTESIAN_POINT('',(-2.1,-0.7,0.6));
#21140=CARTESIAN_POINT('',(-2.1,0.,0.6));
#21141=CARTESIAN_POINT('',(-1.2,-0.7,0.6));
#21142=CARTESIAN_POINT('',(-1.2,-0.7,0.6));
#21143=CARTESIAN_POINT('',(-1.2,0.,0.6));
#21144=CARTESIAN_POINT('',(-1.875,3.36777869765522E-17,0.6));
#21145=CARTESIAN_POINT('Origin',(-1.6,0.,0.6));
#21146=CARTESIAN_POINT('Origin',(-1.2,0.,0.6));
#21147=CARTESIAN_POINT('',(-1.2,-0.7,3.75));
#21148=CARTESIAN_POINT('',(-1.2,-0.7,3.75));
#21149=CARTESIAN_POINT('',(-1.2,0.7,3.75));
#21150=CARTESIAN_POINT('',(-1.2,0.,3.75));
#21151=CARTESIAN_POINT('',(-1.2,0.7,3.75));
#21152=CARTESIAN_POINT('',(-1.2,-2.02066721859313E-17,3.515));
#21153=CARTESIAN_POINT('Origin',(-1.2,0.,3.35));
#21154=CARTESIAN_POINT('Origin',(1.2,0.,0.6));
#21155=CARTESIAN_POINT('',(2.1,-0.7,0.6));
#21156=CARTESIAN_POINT('',(2.1,0.7,0.6));
#21157=CARTESIAN_POINT('',(2.1,0.,0.6));
#21158=CARTESIAN_POINT('',(1.2,0.7,0.6));
#21159=CARTESIAN_POINT('',(2.1,0.7,0.6));
#21160=CARTESIAN_POINT('',(1.2,0.,0.6));
#21161=CARTESIAN_POINT('',(1.2,-0.7,0.6));
#21162=CARTESIAN_POINT('',(1.2,0.,0.6));
#21163=CARTESIAN_POINT('',(2.1,-0.7,0.6));
#21164=CARTESIAN_POINT('',(1.325,3.36777869765522E-17,0.6));
#21165=CARTESIAN_POINT('Origin',(1.6,0.,0.6));
#21166=CARTESIAN_POINT('Origin',(0.1,0.,3.35));
#21167=CARTESIAN_POINT('',(0.1,-2.75545529808155E-17,3.575));
#21168=CARTESIAN_POINT('Origin',(0.1,0.,3.35));
#21169=CARTESIAN_POINT('',(1.2,2.75545529808155E-17,3.575));
#21170=CARTESIAN_POINT('',(0.1,-2.75545529808155E-17,3.575));
#21171=CARTESIAN_POINT('Origin',(1.2,0.,3.35));
#21172=CARTESIAN_POINT('Origin',(0.,0.,3.35));
#21173=CARTESIAN_POINT('',(-0.1,2.02066721859313E-17,3.515));
#21174=CARTESIAN_POINT('',(0.,-2.02066721859313E-17,3.515));
#21175=CARTESIAN_POINT('Origin',(-0.1,0.,3.35));
#21176=CARTESIAN_POINT('Origin',(-1.6,0.,-0.05));
#21177=CARTESIAN_POINT('',(-1.875,-3.36777869765522E-17,0.));
#21178=CARTESIAN_POINT('Origin',(-1.6,0.,0.));
#21179=CARTESIAN_POINT('',(-1.875,-3.36777869765522E-17,-0.05));
#21180=CARTESIAN_POINT('Origin',(1.6,0.,-0.05));
#21181=CARTESIAN_POINT('',(1.325,-3.36777869765522E-17,0.));
#21182=CARTESIAN_POINT('Origin',(1.6,0.,0.));
#21183=CARTESIAN_POINT('',(1.325,-3.36777869765522E-17,-0.05));
#21184=CARTESIAN_POINT('Origin',(0.,0.,2.3));
#21185=CARTESIAN_POINT('',(-0.6,-0.7,2.3));
#21186=CARTESIAN_POINT('Origin',(0.,-0.7,2.3));
#21187=CARTESIAN_POINT('',(-0.6,0.7,2.3));
#21188=CARTESIAN_POINT('',(-0.6,0.,2.3));
#21189=CARTESIAN_POINT('Origin',(0.,0.7,2.3));
#21190=CARTESIAN_POINT('Origin',(0.,-0.7,1.875));
#21191=CARTESIAN_POINT('',(-2.1,-0.7,0.));
#21192=CARTESIAN_POINT('',(-2.1,-0.7,0.6));
#21193=CARTESIAN_POINT('',(2.1,-0.7,0.));
#21194=CARTESIAN_POINT('',(-2.1,-0.7,0.));
#21195=CARTESIAN_POINT('',(2.1,-0.7,0.));
#21196=CARTESIAN_POINT('',(1.2,-0.7,3.75));
#21197=CARTESIAN_POINT('',(1.2,-0.7,0.6));
#21198=CARTESIAN_POINT('',(0.1,-0.7,3.75));
#21199=CARTESIAN_POINT('',(1.2,-0.7,3.75));
#21200=CARTESIAN_POINT('',(0.1,-0.7,2.95));
#21201=CARTESIAN_POINT('',(0.1,-0.7,3.75));
#21202=CARTESIAN_POINT('',(-0.1,-0.7,2.95));
#21203=CARTESIAN_POINT('',(0.1,-0.7,2.95));
#21204=CARTESIAN_POINT('',(-0.1,-0.7,3.75));
#21205=CARTESIAN_POINT('',(-0.1,-0.7,2.95));
#21206=CARTESIAN_POINT('',(-0.1,-0.7,3.75));
#21207=CARTESIAN_POINT('Origin',(-2.1,0.,0.));
#21208=CARTESIAN_POINT('',(-2.1,0.7,0.));
#21209=CARTESIAN_POINT('',(-2.1,0.7,0.6));
#21210=CARTESIAN_POINT('',(-2.1,0.,0.));
#21211=CARTESIAN_POINT('Origin',(2.1,0.,0.));
#21212=CARTESIAN_POINT('',(2.1,0.7,0.));
#21213=CARTESIAN_POINT('',(-2.1,0.7,0.));
#21214=CARTESIAN_POINT('',(2.1,0.,0.));
#21215=CARTESIAN_POINT('Origin',(2.1,0.,0.6));
#21216=CARTESIAN_POINT('',(2.1,0.7,0.));
#21217=CARTESIAN_POINT('Origin',(1.2,0.,3.75));
#21218=CARTESIAN_POINT('',(1.2,0.7,3.75));
#21219=CARTESIAN_POINT('',(1.2,0.7,0.6));
#21220=CARTESIAN_POINT('',(1.2,0.,3.75));
#21221=CARTESIAN_POINT('Origin',(0.1,0.,3.75));
#21222=CARTESIAN_POINT('',(0.1,0.7,3.75));
#21223=CARTESIAN_POINT('',(1.2,0.7,3.75));
#21224=CARTESIAN_POINT('',(0.1,0.,3.75));
#21225=CARTESIAN_POINT('Origin',(0.1,0.,2.95));
#21226=CARTESIAN_POINT('',(0.1,0.7,2.95));
#21227=CARTESIAN_POINT('',(0.1,0.7,3.75));
#21228=CARTESIAN_POINT('',(0.1,0.,2.95));
#21229=CARTESIAN_POINT('Origin',(-0.1,0.,2.95));
#21230=CARTESIAN_POINT('',(-0.1,0.7,2.95));
#21231=CARTESIAN_POINT('',(0.1,0.7,2.95));
#21232=CARTESIAN_POINT('',(-0.1,0.,2.95));
#21233=CARTESIAN_POINT('Origin',(-0.1,0.,3.75));
#21234=CARTESIAN_POINT('',(-0.1,0.7,3.75));
#21235=CARTESIAN_POINT('',(-0.1,0.7,2.95));
#21236=CARTESIAN_POINT('',(-0.1,0.,3.75));
#21237=CARTESIAN_POINT('Origin',(-1.2,0.,3.75));
#21238=CARTESIAN_POINT('',(-0.1,0.7,3.75));
#21239=CARTESIAN_POINT('Origin',(0.,0.7,1.875));
#22329=UNCERTAINTY_MEASURE_WITH_UNIT(LENGTH_MEASURE(0.001),#22395,
'DISTANCE_ACCURACY_VALUE',
'Maximum model space distance between geometric entities at asserted c
onnectivities');
#22343=UNCERTAINTY_MEASURE_WITH_UNIT(LENGTH_MEASURE(0.001),#22395,
'DISTANCE_ACCURACY_VALUE',
'Maximum model space distance between geometric entities at asserted c
onnectivities');
#22380=(
GEOMETRIC_REPRESENTATION_CONTEXT(3)
GLOBAL_UNCERTAINTY_ASSIGNED_CONTEXT((#22329))
GLOBAL_UNIT_ASSIGNED_CONTEXT((#22395,#22397,#22398))
REPRESENTATION_CONTEXT('','3D')
);
#22394=(
GEOMETRIC_REPRESENTATION_CONTEXT(3)
GLOBAL_UNCERTAINTY_ASSIGNED_CONTEXT((#22343))
GLOBAL_UNIT_ASSIGNED_CONTEXT((#22395,#22397,#22398))
REPRESENTATION_CONTEXT('','3D')
);
#22395=(
LENGTH_UNIT()
NAMED_UNIT(*)
SI_UNIT(.CENTI.,.METRE.)
);
#22397=(
NAMED_UNIT(*)
PLANE_ANGLE_UNIT()
SI_UNIT($,.RADIAN.)
);
#22398=(
NAMED_UNIT(*)
SI_UNIT($,.STERADIAN.)
SOLID_ANGLE_UNIT()
);
#22435=SHAPE_DEFINITION_REPRESENTATION(#22485,#22674);
#22485=PRODUCT_DEFINITION_SHAPE('',$,#22725);
#22674=SHAPE_REPRESENTATION('',(#10349),#22380);
#22688=PRODUCT_DEFINITION_CONTEXT('part definition',#22840,'design');
#22725=PRODUCT_DEFINITION('Shaft Support - 12 mm Bore',
'Shaft Support - 12 mm Bore',#22775,#22688);
#22775=PRODUCT_DEFINITION_FORMATION('',$,#22878);
#22840=APPLICATION_CONTEXT(
'Core Data for Automotive Mechanical Design Process');
#22841=PRODUCT_CONTEXT('part definition',#22840,'mechanical');
#22878=PRODUCT('Shaft Support - 12 mm Bore',
'Shaft Support - 12 mm Bore','Shaft Support - 12 mm Bore',(#22841));
#22955=COLOUR_RGB('Grey',0.48,0.52,0.57);
#22956=FILL_AREA_STYLE_COLOUR('',#22955);
#22957=FILL_AREA_STYLE('',(#22956));
#22958=SURFACE_STYLE_FILL_AREA(#22957);
#22959=SURFACE_SIDE_STYLE('',(#22958));
#22960=SURFACE_STYLE_USAGE(.BOTH.,#22959);
#22961=PRESENTATION_STYLE_ASSIGNMENT((#22960));
ENDSEC;
END-ISO-10303-21;
